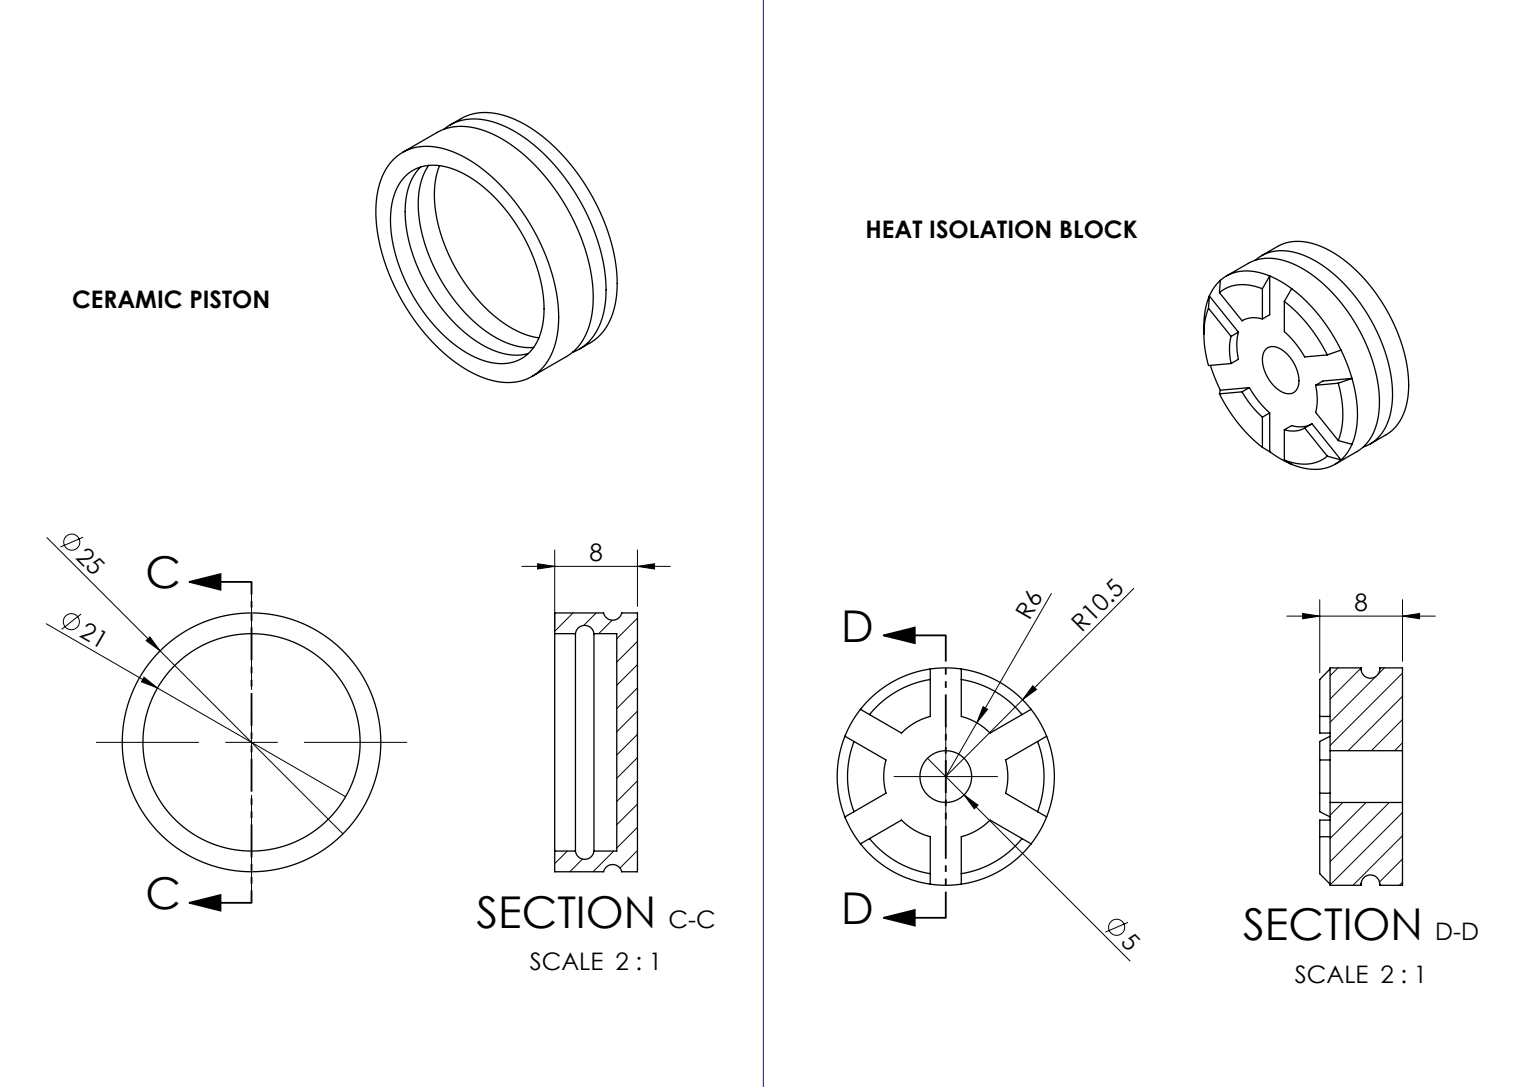
ISO-10303-21;
HEADER;
FILE_DESCRIPTION (('STEP AP214'),
    '1' );
FILE_NAME ('ceramic piston.step',
    '2026-09-24T10:28:59',
    ( '' ),
    ( '' ),
    'SwSTEP 2.0',
    'SolidWorks 2026',
    '' );
FILE_SCHEMA (( 'AUTOMOTIVE_DESIGN' ));
ENDSEC;

DATA;
#112=CARTESIAN_POINT ( 'NONE',  ( 0.000000000000000000, 0.000000000000000000, -4.000000000000000000 ) ) ;
#155=ORIENTED_EDGE ( 'NONE', *, *, #14955, .F. ) ;
#250=CARTESIAN_POINT ( 'NONE',  ( 0.000000000000000000, 0.000000000000000000, -9.600000000000001421 ) ) ;
#253=CARTESIAN_POINT ( 'NONE',  ( 0.000000000000000000, 0.000000000000000000, -9.600000000000001421 ) ) ;
#293=DIRECTION ( 'NONE',  ( 0.9237280213470681067, 0.3830490080632377170, 0.000000000000000000 ) ) ;
#316=CARTESIAN_POINT ( 'NONE',  ( 0.000000000000000000, 0.000000000000000000, -4.000000000000000000 ) ) ;
#333=DIRECTION ( 'NONE',  ( 1.000000000000000000, 0.000000000000000000, -0.000000000000000000 ) ) ;
#391=DIRECTION ( 'NONE',  ( 0.000000000000000000, 0.000000000000000000, 1.000000000000000000 ) ) ;
#452=ORIENTED_EDGE ( 'NONE', *, *, #3011, .F. ) ;
#524=DIRECTION ( 'NONE',  ( 1.000000000000000000, 0.000000000000000000, 0.000000000000000000 ) ) ;
#531=ORIENTED_EDGE ( 'NONE', *, *, #5477, .T. ) ;
#536=VECTOR ( 'NONE', #17608, 1000.000000000000000 ) ;
#599=STYLED_ITEM ( 'NONE', ( #6343 ), #8978 ) ;
#629=ADVANCED_FACE ( 'NONE', ( #5533 ), #13348, .F. ) ;
#659=EDGE_CURVE ( 'NONE', #16901, #17078, #11601, .T. ) ;
#709=ADVANCED_FACE ( 'NONE', ( #11224 ), #11887, .F. ) ;
#714=VERTEX_POINT ( 'NONE', #14072 ) ;
#715=ORIENTED_EDGE ( 'NONE', *, *, #7263, .T. ) ;
#770=CYLINDRICAL_SURFACE ( 'NONE', #14705, 12.50000000000000000 ) ;
#788=PRODUCT_DEFINITION_FORMATION_WITH_SPECIFIED_SOURCE ( 'ANY', '', #8245, .NOT_KNOWN. ) ;
#804=EDGE_CURVE ( 'NONE', #14976, #15476, #12782, .T. ) ;
#811=( NAMED_UNIT ( * ) SI_UNIT ( $, .STERADIAN. ) SOLID_ANGLE_UNIT ( ) );
#858=DIRECTION ( 'NONE',  ( -0.000000000000000000, -0.000000000000000000, -1.000000000000000000 ) ) ;
#922=DIRECTION ( 'NONE',  ( -1.000000000000000000, 0.000000000000000000, 0.000000000000000000 ) ) ;
#925=AXIS2_PLACEMENT_3D ( 'NONE', #16168, #3464, #2298 ) ;
#964=CIRCLE ( 'NONE', #17508, 10.50000000000000000 ) ;
#1034=VERTEX_POINT ( 'NONE', #3000 ) ;
#1048=PRODUCT_DEFINITION ( 'UNKNOWN', '', #788, #12463 ) ;
#1143=ORIENTED_EDGE ( 'NONE', *, *, #6595, .F. ) ;
#1148=VECTOR ( 'NONE', #6040, 1000.000000000000000 ) ;
#1152=CARTESIAN_POINT ( 'NONE',  ( 11.73134587110777005, 4.864722402403120149, -9.600000000000001421 ) ) ;
#1158=VERTEX_POINT ( 'NONE', #9063 ) ;
#1172=AXIS2_PLACEMENT_3D ( 'NONE', #8228, #13759, #1339 ) ;
#1199=CARTESIAN_POINT ( 'NONE',  ( 0.000000000000000000, 0.000000000000000000, -4.000000000000000000 ) ) ;
#1261=DIRECTION ( 'NONE',  ( 0.000000000000000000, 0.000000000000000000, 1.000000000000000000 ) ) ;
#1315=ORIENTED_EDGE ( 'NONE', *, *, #13930, .F. ) ;
#1339=DIRECTION ( 'NONE',  ( 1.000000000000000000, 0.000000000000000000, 0.000000000000000000 ) ) ;
#1365=CARTESIAN_POINT ( 'NONE',  ( 0.000000000000000000, 0.000000000000000000, -10.00000000000000000 ) ) ;
#1438=AXIS2_PLACEMENT_3D ( 'NONE', #2614, #17876, #10918 ) ;
#1444=CIRCLE ( 'NONE', #7818, 12.50000000000000000 ) ;
#1469=COLOUR_RGB ( '', 0.72549020, 0.75294118, 0.79215686) ;
#1475=EDGE_LOOP ( 'NONE', ( #10011, #4500, #155, #17294, #7332 ) ) ;
#1495=CYLINDRICAL_SURFACE ( 'NONE', #12703, 10.50000000000000000 ) ;
#1505=TOROIDAL_SURFACE ( 'NONE', #14826, 10.40000000000000036, 0.9000000000000003553 ) ;
#1527=DIRECTION ( 'NONE',  ( 1.000000000000000000, 0.000000000000000000, 0.000000000000000000 ) ) ;
#1538=ADVANCED_FACE ( 'NONE', ( #6383 ), #1505, .F. ) ;
#1541=CIRCLE ( 'NONE', #11662, 10.50000000000000000 ) ;
#1555=ORIENTED_EDGE ( 'NONE', *, *, #12558, .F. ) ;
#1556=AXIS2_PLACEMENT_3D ( 'NONE', #12533, #15688, #5624 ) ;
#1570=VERTEX_POINT ( 'NONE', #6290 ) ;
#1706=FACE_OUTER_BOUND ( 'NONE', #10911, .T. ) ;
#1743=ADVANCED_FACE ( 'NONE', ( #15891 ), #14883, .T. ) ;
#1830=LINE ( 'NONE', #17063, #3240 ) ;
#1846=EDGE_CURVE ( 'NONE', #16993, #17950, #4103, .T. ) ;
#1863=AXIS2_PLACEMENT_3D ( 'NONE', #15659, #6311, #2165 ) ;
#1877=CARTESIAN_POINT ( 'NONE',  ( 12.50000000000000000, 1.530808498934191521E-15, -10.47749643873921244 ) ) ;
#1897=CARTESIAN_POINT ( 'NONE',  ( 0.000000000000000000, 0.000000000000000000, -12.00000000000000000 ) ) ;
#1937=EDGE_CURVE ( 'NONE', #16345, #6066, #10175, .T. ) ;
#1962=DIRECTION ( 'NONE',  ( -5.026720092345836698E-22, 4.581671729415424240E-22, -1.000000000000000000 ) ) ;
#1978=ORIENTED_EDGE ( 'NONE', *, *, #804, .F. ) ;
#2009=AXIS2_PLACEMENT_3D ( 'NONE', #10405, #10657, #10838 ) ;
#2016=EDGE_LOOP ( 'NONE', ( #5308, #3767, #12168, #12352, #15309 ) ) ;
#2054=CIRCLE ( 'NONE', #4054, 10.50000000000000000 ) ;
#2086=ORIENTED_EDGE ( 'NONE', *, *, #12227, .F. ) ;
#2089=VERTEX_POINT ( 'NONE', #7177 ) ;
#2101=EDGE_CURVE ( 'NONE', #9766, #6169, #5832, .T. ) ;
#2103=( NAMED_UNIT ( * ) PLANE_ANGLE_UNIT ( ) SI_UNIT ( $, .RADIAN. ) );
#2146=EDGE_CURVE ( 'NONE', #9766, #2089, #1830, .T. ) ;
#2165=DIRECTION ( 'NONE',  ( -1.000000000000000000, 0.000000000000000000, 0.000000000000000000 ) ) ;
#2195=( NAMED_UNIT ( * ) PLANE_ANGLE_UNIT ( ) SI_UNIT ( $, .RADIAN. ) );
#2230=DIRECTION ( 'NONE',  ( 5.026720092345836698E-22, -4.581671729415424240E-22, 1.000000000000000000 ) ) ;
#2298=DIRECTION ( 'NONE',  ( -1.000000000000000000, 0.000000000000000000, 0.000000000000000000 ) ) ;
#2338=CARTESIAN_POINT ( 'NONE',  ( 0.000000000000000000, 0.000000000000000000, -4.000000000000000000 ) ) ;
#2471=EDGE_CURVE ( 'NONE', #1158, #1034, #7607, .T. ) ;
#2482=CARTESIAN_POINT ( 'NONE',  ( 0.000000000000000000, 0.000000000000000000, -10.00000000000000000 ) ) ;
#2494=SURFACE_STYLE_FILL_AREA ( #4027 ) ;
#2598=DIRECTION ( 'NONE',  ( 0.9237280213470682178, 0.3830490080632377170, 0.000000000000000000 ) ) ;
#2613=DIRECTION ( 'NONE',  ( -0.3830490080632376615, 0.9237280213470682178, 0.000000000000000000 ) ) ;
#2614=CARTESIAN_POINT ( 'NONE',  ( 0.000000000000000000, 0.000000000000000000, -9.600000000000001421 ) ) ;
#2623=ADVANCED_FACE ( 'NONE', ( #12156 ), #5002, .T. ) ;
#2627=STYLED_ITEM ( 'NONE', ( #17931 ), #11433 ) ;
#2632=AXIS2_PLACEMENT_3D ( 'NONE', #112, #391, #5897 ) ;
#2684=AXIS2_PLACEMENT_3D ( 'NONE', #253, #10021, #16757 ) ;
#2690=EDGE_CURVE ( 'NONE', #6877, #15184, #9894, .T. ) ;
#2691=CARTESIAN_POINT ( 'NONE',  ( 10.50000000000000000, 1.285879139104720831E-15, -4.000000000000000000 ) ) ;
#2706=DIRECTION ( 'NONE',  ( -1.000000000000000000, 0.000000000000000000, 0.000000000000000000 ) ) ;
#2741=LINE ( 'NONE', #8262, #13559 ) ;
#2764=SURFACE_STYLE_USAGE ( .BOTH. , #8017 ) ;
#2788=ADVANCED_FACE ( 'NONE', ( #9518 ), #16296, .F. ) ;
#2793=CARTESIAN_POINT ( 'NONE',  ( -11.54660026683835383, -4.788112600790469742, -10.47749643873921244 ) ) ;
#2837=ORIENTED_EDGE ( 'NONE', *, *, #804, .T. ) ;
#2900=( GEOMETRIC_REPRESENTATION_CONTEXT ( 3 ) GLOBAL_UNCERTAINTY_ASSIGNED_CONTEXT ( ( #12605 ) ) GLOBAL_UNIT_ASSIGNED_CONTEXT ( ( #13555, #12455, #3862 ) ) REPRESENTATION_CONTEXT ( 'NONE', 'WORKASPACE' ) );
#2946=DIRECTION ( 'NONE',  ( 1.000000000000000000, -4.440892098500626162E-15, 0.000000000000000000 ) ) ;
#3000=CARTESIAN_POINT ( 'NONE',  ( 11.54660026683835206, 4.788112600790471518, -10.47749643873921244 ) ) ;
#3011=EDGE_CURVE ( 'NONE', #15476, #16993, #13400, .T. ) ;
#3190=EDGE_LOOP ( 'NONE', ( #4795, #17103, #11231, #9291, #13094, #3504 ) ) ;
#3233=ORIENTED_EDGE ( 'NONE', *, *, #17773, .F. ) ;
#3240=VECTOR ( 'NONE', #6438, 1000.000000000000000 ) ;
#3256=ORIENTED_EDGE ( 'NONE', *, *, #16158, .T. ) ;
#3285=FACE_OUTER_BOUND ( 'NONE', #8751, .T. ) ;
#3349=CARTESIAN_POINT ( 'NONE',  ( 11.54660026683835206, 4.788112600790471518, -8.722503561260788629 ) ) ;
#3358=CARTESIAN_POINT ( 'NONE',  ( 8.472608240843633681E-22, -7.722472891792491889E-22, -7.794427190999915211 ) ) ;
#3382=CARTESIAN_POINT ( 'NONE',  ( -10.89999065189540772, -4.519978295146205305, -9.600000000000001421 ) ) ;
#3393=CIRCLE ( 'NONE', #8898, 12.50000000000000000 ) ;
#3430=AXIS2_PLACEMENT_3D ( 'NONE', #1199, #10952, #8080 ) ;
#3464=DIRECTION ( 'NONE',  ( -0.000000000000000000, -0.000000000000000000, -1.000000000000000000 ) ) ;
#3504=ORIENTED_EDGE ( 'NONE', *, *, #6011, .T. ) ;
#3531=AXIS2_PLACEMENT_3D ( 'NONE', #2482, #10701, #17662 ) ;
#3556=EDGE_CURVE ( 'NONE', #17384, #13349, #3393, .T. ) ;
#3575=AXIS2_PLACEMENT_3D ( 'NONE', #5095, #17575, #9272 ) ;
#3606=ORIENTED_EDGE ( 'NONE', *, *, #9596, .T. ) ;
#3640=VERTEX_POINT ( 'NONE', #3382 ) ;
#3750=AXIS2_PLACEMENT_3D ( 'NONE', #10192, #1962, #10363 ) ;
#3767=ORIENTED_EDGE ( 'NONE', *, *, #5434, .T. ) ;
#3784=( GEOMETRIC_REPRESENTATION_CONTEXT ( 3 ) GLOBAL_UNCERTAINTY_ASSIGNED_CONTEXT ( ( #4445 ) ) GLOBAL_UNIT_ASSIGNED_CONTEXT ( ( #13509, #2103, #811 ) ) REPRESENTATION_CONTEXT ( 'NONE', 'WORKASPACE' ) );
#3793=ORIENTED_EDGE ( 'NONE', *, *, #2471, .T. ) ;
#3840=CIRCLE ( 'NONE', #8463, 0.9000000000000011324 ) ;
#3849=DIRECTION ( 'NONE',  ( -0.9979201627913402151, 0.06446199418653550395, 5.311609029246448998E-22 ) ) ;
#3860=ORIENTED_EDGE ( 'NONE', *, *, #2101, .T. ) ;
#3862=( NAMED_UNIT ( * ) SI_UNIT ( $, .STERADIAN. ) SOLID_ANGLE_UNIT ( ) );
#3888=DIRECTION ( 'NONE',  ( -0.000000000000000000, -0.000000000000000000, -1.000000000000000000 ) ) ;
#3911=CARTESIAN_POINT ( 'NONE',  ( 0.000000000000000000, 0.000000000000000000, -8.722503561260788629 ) ) ;
#3924=EDGE_CURVE ( 'NONE', #6169, #8696, #9457, .T. ) ;
#3984=ADVANCED_FACE ( 'NONE', ( #16284 ), #770, .T. ) ;
#4010=CIRCLE ( 'NONE', #10365, 0.9000000000000011324 ) ;
#4024=CARTESIAN_POINT ( 'NONE',  ( 0.000000000000000000, 0.000000000000000000, -8.722503561260788629 ) ) ;
#4027=FILL_AREA_STYLE ('',( #16293 ) ) ;
#4054=AXIS2_PLACEMENT_3D ( 'NONE', #8842, #15368, #5926 ) ;
#4057=CARTESIAN_POINT ( 'NONE',  ( 0.000000000000000000, 0.000000000000000000, -4.000000000000000000 ) ) ;
#4097=CIRCLE ( 'NONE', #17745, 0.9000000000000003553 ) ;
#4103=CIRCLE ( 'NONE', #9881, 10.50000000000000000 ) ;
#4195=CARTESIAN_POINT ( 'NONE',  ( 0.000000000000000000, 0.000000000000000000, -9.600000000000001421 ) ) ;
#4276=ORIENTED_EDGE ( 'NONE', *, *, #5477, .F. ) ;
#4308=DIRECTION ( 'NONE',  ( 1.000000000000000000, 0.000000000000000000, 0.000000000000000000 ) ) ;
#4339=ORIENTED_EDGE ( 'NONE', *, *, #5350, .T. ) ;
#4393=EDGE_LOOP ( 'NONE', ( #8466, #15017, #11576, #7109, #5872 ) ) ;
#4424=DIRECTION ( 'NONE',  ( 0.000000000000000000, 0.000000000000000000, 1.000000000000000000 ) ) ;
#4432=CIRCLE ( 'NONE', #11963, 10.50000000000000000 ) ;
#4445=UNCERTAINTY_MEASURE_WITH_UNIT (LENGTH_MEASURE( 1.000000000000000082E-05 ), #13509, 'distance_accuracy_value', 'NONE');
#4491=FACE_OUTER_BOUND ( 'NONE', #10765, .T. ) ;
#4495=CARTESIAN_POINT ( 'NONE',  ( -10.47816170930907553, 0.6768509389586230274, -7.794427190999915211 ) ) ;
#4500=ORIENTED_EDGE ( 'NONE', *, *, #8547, .T. ) ;
#4630=PLANE ( 'NONE',  #16310 ) ;
#4653=DIRECTION ( 'NONE',  ( -1.000000000000000000, -1.065814103640150279E-14, 0.000000000000000000 ) ) ;
#4720=EDGE_CURVE ( 'NONE', #714, #6066, #17381, .T. ) ;
#4795=ORIENTED_EDGE ( 'NONE', *, *, #12262, .F. ) ;
#4811=APPLICATION_CONTEXT ( 'automotive_design' ) ;
#4924=CARTESIAN_POINT ( 'NONE',  ( 1.746467850512308208E-21, -1.591841644184202181E-21, -6.005572809000082835 ) ) ;
#5002=CYLINDRICAL_SURFACE ( 'NONE', #7017, 12.50000000000000000 ) ;
#5095=CARTESIAN_POINT ( 'NONE',  ( 0.000000000000000000, 0.000000000000000000, 0.000000000000000000 ) ) ;
#5116=CARTESIAN_POINT ( 'NONE',  ( 12.50000000000000000, 1.530808498934191521E-15, -4.000000000000000000 ) ) ;
#5148=SURFACE_STYLE_FILL_AREA ( #6606 ) ;
#5160=DIRECTION ( 'NONE',  ( 0.06446199418653537905, 0.9979201627913403261, 4.248110196704583871E-22 ) ) ;
#5184=PLANE ( 'NONE',  #3531 ) ;
#5252=AXIS2_PLACEMENT_3D ( 'NONE', #1365, #6890, #12419 ) ;
#5261=DIRECTION ( 'NONE',  ( -0.9979201627913402151, 0.06446199418653550395, 5.311609029246448998E-22 ) ) ;
#5267=AXIS2_PLACEMENT_3D ( 'NONE', #9775, #6898, #16518 ) ;
#5308=ORIENTED_EDGE ( 'NONE', *, *, #8547, .F. ) ;
#5350=EDGE_CURVE ( 'NONE', #1158, #3640, #14742, .T. ) ;
#5434=EDGE_CURVE ( 'NONE', #3640, #6169, #4010, .T. ) ;
#5457=AXIS2_PLACEMENT_3D ( 'NONE', #9421, #8920, #4653 ) ;
#5477=EDGE_CURVE ( 'NONE', #17078, #16901, #8353, .T. ) ;
#5533=FACE_OUTER_BOUND ( 'NONE', #2016, .T. ) ;
#5539=CIRCLE ( 'NONE', #17468, 0.9000000000000011324 ) ;
#5554=AXIS2_PLACEMENT_3D ( 'NONE', #8563, #16731, #2946 ) ;
#5624=DIRECTION ( 'NONE',  ( -1.000000000000000000, 0.000000000000000000, 0.000000000000000000 ) ) ;
#5636=ORIENTED_EDGE ( 'NONE', *, *, #6443, .F. ) ;
#5643=LINE ( 'NONE', #8651, #15902 ) ;
#5706=ORIENTED_EDGE ( 'NONE', *, *, #8457, .T. ) ;
#5756=ORIENTED_EDGE ( 'NONE', *, *, #16630, .T. ) ;
#5763=CARTESIAN_POINT ( 'NONE',  ( -10.47816170930907553, 0.6768509389586230274, -6.005572809000082835 ) ) ;
#5802=CIRCLE ( 'NONE', #12188, 12.50000000000000000 ) ;
#5832=CIRCLE ( 'NONE', #8171, 12.50000000000000000 ) ;
#5835=PRODUCT_CONTEXT ( 'NONE', #13620, 'mechanical' ) ;
#5872=ORIENTED_EDGE ( 'NONE', *, *, #9666, .F. ) ;
#5897=DIRECTION ( 'NONE',  ( 1.000000000000000000, 0.000000000000000000, 0.000000000000000000 ) ) ;
#5918=DIRECTION ( 'NONE',  ( 0.9979201627913403261, -0.06446199418653547619, 0.000000000000000000 ) ) ;
#5926=DIRECTION ( 'NONE',  ( 1.000000000000000000, 0.000000000000000000, 0.000000000000000000 ) ) ;
#5953=ADVANCED_FACE ( 'NONE', ( #6627 ), #16356, .F. ) ;
#6011=EDGE_CURVE ( 'NONE', #13121, #11972, #7798, .T. ) ;
#6025=ORIENTED_EDGE ( 'NONE', *, *, #9596, .F. ) ;
#6030=FACE_OUTER_BOUND ( 'NONE', #15171, .T. ) ;
#6040=DIRECTION ( 'NONE',  ( -0.000000000000000000, -0.000000000000000000, -1.000000000000000000 ) ) ;
#6066=VERTEX_POINT ( 'NONE', #7458 ) ;
#6140=CARTESIAN_POINT ( 'NONE',  ( -12.50000000000000000, 0.000000000000000000, -4.000000000000000000 ) ) ;
#6165=CARTESIAN_POINT ( 'NONE',  ( -12.50000000000000000, 0.000000000000000000, -10.47749643873921244 ) ) ;
#6169=VERTEX_POINT ( 'NONE', #2793 ) ;
#6235=EDGE_CURVE ( 'NONE', #1570, #2089, #17079, .T. ) ;
#6254=( LENGTH_UNIT ( ) NAMED_UNIT ( * ) SI_UNIT ( .MILLI., .METRE. ) );
#6290=CARTESIAN_POINT ( 'NONE',  ( -12.50000000000000000, 0.000000000000000000, -12.00000000000000000 ) ) ;
#6311=DIRECTION ( 'NONE',  ( -0.000000000000000000, -0.000000000000000000, -1.000000000000000000 ) ) ;
#6343=PRESENTATION_STYLE_ASSIGNMENT (( #6528 ) ) ;
#6383=FACE_OUTER_BOUND ( 'NONE', #3190, .T. ) ;
#6438=DIRECTION ( 'NONE',  ( -0.000000000000000000, -0.000000000000000000, -1.000000000000000000 ) ) ;
#6443=EDGE_CURVE ( 'NONE', #8696, #1570, #5643, .T. ) ;
#6457=CARTESIAN_POINT ( 'NONE',  ( 10.37836969302994028, -0.6704047395399680420, -6.899999999999998579 ) ) ;
#6465=DIRECTION ( 'NONE',  ( 1.000000000000000000, 0.000000000000000000, 0.000000000000000000 ) ) ;
#6509=ADVANCED_FACE ( 'NONE', ( #16821 ), #1495, .F. ) ;
#6528=SURFACE_STYLE_USAGE ( .BOTH. , #12043 ) ;
#6540=DIRECTION ( 'NONE',  ( 0.000000000000000000, 0.000000000000000000, 1.000000000000000000 ) ) ;
#6541=DIRECTION ( 'NONE',  ( 0.3830490080632377725, -0.9237280213470682178, 0.000000000000000000 ) ) ;
#6595=EDGE_CURVE ( 'NONE', #15658, #16993, #9799, .T. ) ;
#6606=FILL_AREA_STYLE ('',( #16068 ) ) ;
#6627=FACE_OUTER_BOUND ( 'NONE', #4393, .T. ) ;
#6712=CARTESIAN_POINT ( 'NONE',  ( 1.746467850512308208E-21, -1.591841644184202181E-21, -6.005572809000082835 ) ) ;
#6719=CARTESIAN_POINT ( 'NONE',  ( 10.50000000000000000, 1.285879139104720831E-15, -7.794427190999915211 ) ) ;
#6731=CIRCLE ( 'NONE', #14277, 0.9000000000000003553 ) ;
#6794=VERTEX_POINT ( 'NONE', #8518 ) ;
#6877=VERTEX_POINT ( 'NONE', #3349 ) ;
#6890=DIRECTION ( 'NONE',  ( 0.000000000000000000, 0.000000000000000000, 1.000000000000000000 ) ) ;
#6898=DIRECTION ( 'NONE',  ( 0.000000000000000000, 0.000000000000000000, 1.000000000000000000 ) ) ;
#7017=AXIS2_PLACEMENT_3D ( 'NONE', #17650, #11798, #14721 ) ;
#7109=ORIENTED_EDGE ( 'NONE', *, *, #4720, .F. ) ;
#7135=DIRECTION ( 'NONE',  ( 0.000000000000000000, 0.000000000000000000, 1.000000000000000000 ) ) ;
#7177=CARTESIAN_POINT ( 'NONE',  ( 12.50000000000000000, 1.530808498934191521E-15, -12.00000000000000000 ) ) ;
#7204=DIRECTION ( 'NONE',  ( 0.000000000000000000, 0.000000000000000000, 1.000000000000000000 ) ) ;
#7219=ADVANCED_FACE ( 'NONE', ( #16405 ), #15036, .F. ) ;
#7224=PLANE ( 'NONE',  #13964 ) ;
#7242=ADVANCED_FACE ( 'NONE', ( #9568 ), #15026, .T. ) ;
#7263=EDGE_CURVE ( 'NONE', #2089, #1570, #16493, .T. ) ;
#7273=COLOUR_RGB ( '', 0.72549020, 0.75294118, 0.79215686) ;
#7279=CARTESIAN_POINT ( 'NONE',  ( 0.000000000000000000, 0.000000000000000000, -4.000000000000000000 ) ) ;
#7332=ORIENTED_EDGE ( 'NONE', *, *, #3556, .F. ) ;
#7375=DIRECTION ( 'NONE',  ( 0.000000000000000000, 0.000000000000000000, 1.000000000000000000 ) ) ;
#7454=CARTESIAN_POINT ( 'NONE',  ( 10.47816170930907553, -0.6768509389586216951, -7.794427190999915211 ) ) ;
#7458=CARTESIAN_POINT ( 'NONE',  ( -10.50000000000000000, 0.000000000000000000, -10.00000000000000000 ) ) ;
#7476=ORIENTED_EDGE ( 'NONE', *, *, #1846, .T. ) ;
#7507=LINE ( 'NONE', #6140, #1148 ) ;
#7517=EDGE_CURVE ( 'NONE', #16901, #13349, #17597, .T. ) ;
#7541=VECTOR ( 'NONE', #13295, 1000.000000000000000 ) ;
#7569=CARTESIAN_POINT ( 'NONE',  ( -10.37836969302994028, 0.6704047395399693743, -6.899999999999998579 ) ) ;
#7585=AXIS2_PLACEMENT_3D ( 'NONE', #11276, #8311, #11182 ) ;
#7607=CIRCLE ( 'NONE', #7891, 0.9000000000000011324 ) ;
#7740=ORIENTED_EDGE ( 'NONE', *, *, #2146, .T. ) ;
#7744=DIRECTION ( 'NONE',  ( -1.000000000000000000, 0.000000000000000000, 0.000000000000000000 ) ) ;
#7780=ORIENTED_EDGE ( 'NONE', *, *, #7517, .F. ) ;
#7798=CIRCLE ( 'NONE', #15320, 10.50000000000000000 ) ;
#7818=AXIS2_PLACEMENT_3D ( 'NONE', #11359, #16928, #4308 ) ;
#7880=EDGE_LOOP ( 'NONE', ( #17660, #1978 ) ) ;
#7891=AXIS2_PLACEMENT_3D ( 'NONE', #9169, #6541, #13343 ) ;
#7946=EDGE_LOOP ( 'NONE', ( #11758, #4339, #1555, #2086, #11320 ) ) ;
#7961=ORIENTED_EDGE ( 'NONE', *, *, #7517, .T. ) ;
#7968=CARTESIAN_POINT ( 'NONE',  ( -11.73134587110777005, -4.864722402403119261, -9.600000000000001421 ) ) ;
#7979=EDGE_LOOP ( 'NONE', ( #7780, #4276, #17656, #14589, #16002 ) ) ;
#7993=CARTESIAN_POINT ( 'NONE',  ( 8.472608240843633681E-22, -7.722472891792491889E-22, -7.794427190999915211 ) ) ;
#8010=DIRECTION ( 'NONE',  ( -1.000000000000000000, 0.000000000000000000, 0.000000000000000000 ) ) ;
#8017=SURFACE_SIDE_STYLE ('',( #2494 ) ) ;
#8080=DIRECTION ( 'NONE',  ( -1.000000000000000000, 0.000000000000000000, 0.000000000000000000 ) ) ;
#8125=DIRECTION ( 'NONE',  ( 0.3830490080632377725, -0.9237280213470682178, 0.000000000000000000 ) ) ;
#8141=CARTESIAN_POINT ( 'NONE',  ( 0.000000000000000000, 0.000000000000000000, -4.000000000000000000 ) ) ;
#8171=AXIS2_PLACEMENT_3D ( 'NONE', #11493, #8803, #11305 ) ;
#8228=CARTESIAN_POINT ( 'NONE',  ( 0.000000000000000000, 0.000000000000000000, -12.00000000000000000 ) ) ;
#8245=PRODUCT ( 'ceramic piston', 'ceramic piston', '', ( #5835 ) ) ;
#8262=CARTESIAN_POINT ( 'NONE',  ( 10.50000000000000000, 1.285879139104720831E-15, -4.000000000000000000 ) ) ;
#8311=DIRECTION ( 'NONE',  ( 0.000000000000000000, 0.000000000000000000, 1.000000000000000000 ) ) ;
#8353=CIRCLE ( 'NONE', #8931, 12.50000000000000000 ) ;
#8457=EDGE_CURVE ( 'NONE', #15476, #14976, #1541, .T. ) ;
#8463=AXIS2_PLACEMENT_3D ( 'NONE', #1152, #8125, #2598 ) ;
#8466=ORIENTED_EDGE ( 'NONE', *, *, #6011, .F. ) ;
#8470=DIRECTION ( 'NONE',  ( -1.000000000000000000, 0.000000000000000000, 0.000000000000000000 ) ) ;
#8485=CARTESIAN_POINT ( 'NONE',  ( 0.000000000000000000, 0.000000000000000000, -12.00000000000000000 ) ) ;
#8518=CARTESIAN_POINT ( 'NONE',  ( 10.50000000000000000, 1.285879139104720831E-15, -6.005572809000082835 ) ) ;
#8539=DIRECTION ( 'NONE',  ( 0.9237280213470681067, 0.3830490080632377170, 0.000000000000000000 ) ) ;
#8547=EDGE_CURVE ( 'NONE', #3640, #1158, #13691, .T. ) ;
#8563=CARTESIAN_POINT ( 'NONE',  ( 0.000000000000000000, 0.000000000000000000, -10.47749643873921244 ) ) ;
#8625=CYLINDRICAL_SURFACE ( 'NONE', #11968, 10.50000000000000000 ) ;
#8651=CARTESIAN_POINT ( 'NONE',  ( -12.50000000000000000, 0.000000000000000000, -4.000000000000000000 ) ) ;
#8696=VERTEX_POINT ( 'NONE', #6165 ) ;
#8709=MECHANICAL_DESIGN_GEOMETRIC_PRESENTATION_REPRESENTATION('',(#2627),#2900);
#8725=FACE_OUTER_BOUND ( 'NONE', #10604, .T. ) ;
#8746=EDGE_CURVE ( 'NONE', #16745, #13121, #4432, .T. ) ;
#8751=EDGE_LOOP ( 'NONE', ( #17194, #2837, #12747, #1143, #12287 ) ) ;
#8803=DIRECTION ( 'NONE',  ( -0.000000000000000000, -0.000000000000000000, -1.000000000000000000 ) ) ;
#8816=DIRECTION ( 'NONE',  ( -0.000000000000000000, -0.000000000000000000, -1.000000000000000000 ) ) ;
#8842=CARTESIAN_POINT ( 'NONE',  ( 8.472608240843633681E-22, -7.722472891792491889E-22, -7.794427190999915211 ) ) ;
#8877=ORIENTED_EDGE ( 'NONE', *, *, #5350, .F. ) ;
#8898=AXIS2_PLACEMENT_3D ( 'NONE', #4024, #7204, #12449 ) ;
#8920=DIRECTION ( 'NONE',  ( 5.026720092345836698E-22, -4.581671729415424240E-22, 1.000000000000000000 ) ) ;
#8931=AXIS2_PLACEMENT_3D ( 'NONE', #8141, #1261, #1527 ) ;
#8978=ADVANCED_BREP_SHAPE_REPRESENTATION ( '', ( #11433, #3575 ), #3784 ) ;
#9063=CARTESIAN_POINT ( 'NONE',  ( 10.89999065189540772, 4.519978295146206193, -9.600000000000001421 ) ) ;
#9071=SHAPE_REPRESENTATION_RELATIONSHIP ( 'NONE' , 'NONE' ,  #16332, #8978 ) ;
#9126=DIRECTION ( 'NONE',  ( 0.000000000000000000, 0.000000000000000000, 1.000000000000000000 ) ) ;
#9169=CARTESIAN_POINT ( 'NONE',  ( 11.73134587110777005, 4.864722402403120149, -9.600000000000001421 ) ) ;
#9172=UNCERTAINTY_MEASURE_WITH_UNIT (LENGTH_MEASURE( 1.000000000000000082E-05 ), #6254, 'distance_accuracy_value', 'NONE');
#9180=EDGE_CURVE ( 'NONE', #17078, #15184, #7507, .T. ) ;
#9272=DIRECTION ( 'NONE',  ( 1.000000000000000000, 0.000000000000000000, 0.000000000000000000 ) ) ;
#9275=( GEOMETRIC_REPRESENTATION_CONTEXT ( 3 ) GLOBAL_UNCERTAINTY_ASSIGNED_CONTEXT ( ( #9172 ) ) GLOBAL_UNIT_ASSIGNED_CONTEXT ( ( #6254, #2195, #15970 ) ) REPRESENTATION_CONTEXT ( 'NONE', 'WORKASPACE' ) );
#9291=ORIENTED_EDGE ( 'NONE', *, *, #17773, .T. ) ;
#9421=CARTESIAN_POINT ( 'NONE',  ( 1.746467850512308208E-21, -1.591841644184202181E-21, -6.005572809000082835 ) ) ;
#9423=CARTESIAN_POINT ( 'NONE',  ( 0.000000000000000000, 0.000000000000000000, -4.000000000000000000 ) ) ;
#9457=CIRCLE ( 'NONE', #10888, 12.50000000000000000 ) ;
#9518=FACE_OUTER_BOUND ( 'NONE', #11290, .T. ) ;
#9568=FACE_OUTER_BOUND ( 'NONE', #10087, .T. ) ;
#9596=EDGE_CURVE ( 'NONE', #8696, #1034, #1444, .T. ) ;
#9666=EDGE_CURVE ( 'NONE', #11972, #714, #2054, .T. ) ;
#9672=EDGE_LOOP ( 'NONE', ( #13955, #12949, #1315, #10879, #13886 ) ) ;
#9680=DIRECTION ( 'NONE',  ( 0.000000000000000000, 0.000000000000000000, 1.000000000000000000 ) ) ;
#9766=VERTEX_POINT ( 'NONE', #1877 ) ;
#9775=CARTESIAN_POINT ( 'NONE',  ( 0.000000000000000000, 0.000000000000000000, -8.722503561260788629 ) ) ;
#9799=CIRCLE ( 'NONE', #5457, 10.50000000000000000 ) ;
#9879=CARTESIAN_POINT ( 'NONE',  ( -12.50000000000000000, 0.000000000000000000, -4.000000000000000000 ) ) ;
#9881=AXIS2_PLACEMENT_3D ( 'NONE', #6712, #13612, #16512 ) ;
#9894=CIRCLE ( 'NONE', #5267, 12.50000000000000000 ) ;
#9902=DIRECTION ( 'NONE',  ( -0.000000000000000000, -0.000000000000000000, -1.000000000000000000 ) ) ;
#9944=ORIENTED_EDGE ( 'NONE', *, *, #12597, .T. ) ;
#10011=ORIENTED_EDGE ( 'NONE', *, *, #12558, .T. ) ;
#10021=DIRECTION ( 'NONE',  ( 0.000000000000000000, 0.000000000000000000, 1.000000000000000000 ) ) ;
#10087=EDGE_LOOP ( 'NONE', ( #16850, #3860, #17086, #11688, #14910 ) ) ;
#10175=CIRCLE ( 'NONE', #5252, 10.50000000000000000 ) ;
#10192=CARTESIAN_POINT ( 'NONE',  ( 8.472608240843633681E-22, -7.722472891792491889E-22, -7.794427190999915211 ) ) ;
#10336=ORIENTED_EDGE ( 'NONE', *, *, #1937, .T. ) ;
#10355=DIRECTION ( 'NONE',  ( -0.06446199418653550395, -0.9979201627913403261, -4.248110196704583871E-22 ) ) ;
#10363=DIRECTION ( 'NONE',  ( 1.000000000000000000, 0.000000000000000000, 0.000000000000000000 ) ) ;
#10365=AXIS2_PLACEMENT_3D ( 'NONE', #7968, #2613, #17706 ) ;
#10380=CYLINDRICAL_SURFACE ( 'NONE', #1863, 10.50000000000000000 ) ;
#10405=CARTESIAN_POINT ( 'NONE',  ( 0.000000000000000000, 0.000000000000000000, -9.600000000000001421 ) ) ;
#10498=CARTESIAN_POINT ( 'NONE',  ( 10.50000000000000000, 1.285879139104720831E-15, -4.000000000000000000 ) ) ;
#10589=CARTESIAN_POINT ( 'NONE',  ( 1.746467850512308208E-21, -1.591841644184202181E-21, -6.005572809000082835 ) ) ;
#10604=EDGE_LOOP ( 'NONE', ( #531, #11943 ) ) ;
#10623=CARTESIAN_POINT ( 'NONE',  ( 0.000000000000000000, 0.000000000000000000, -10.47749643873921244 ) ) ;
#10657=DIRECTION ( 'NONE',  ( 0.000000000000000000, 0.000000000000000000, 1.000000000000000000 ) ) ;
#10659=CARTESIAN_POINT ( 'NONE',  ( -11.73134587110777005, -4.864722402403119261, -9.600000000000001421 ) ) ;
#10701=DIRECTION ( 'NONE',  ( 0.000000000000000000, 0.000000000000000000, 1.000000000000000000 ) ) ;
#10765=EDGE_LOOP ( 'NONE', ( #15447, #17309 ) ) ;
#10838=DIRECTION ( 'NONE',  ( 1.000000000000000000, 0.000000000000000000, 0.000000000000000000 ) ) ;
#10879=ORIENTED_EDGE ( 'NONE', *, *, #4720, .T. ) ;
#10888=AXIS2_PLACEMENT_3D ( 'NONE', #10623, #16196, #11819 ) ;
#10911=EDGE_LOOP ( 'NONE', ( #8877, #3793, #6025, #14457, #11378 ) ) ;
#10918=DIRECTION ( 'NONE',  ( 0.9237280213470681067, 0.3830490080632377170, 0.000000000000000000 ) ) ;
#10952=DIRECTION ( 'NONE',  ( -0.000000000000000000, -0.000000000000000000, -1.000000000000000000 ) ) ;
#11031=AXIS2_PLACEMENT_3D ( 'NONE', #250, #16486, #13761 ) ;
#11057=CARTESIAN_POINT ( 'NONE',  ( 12.50000000000000000, 1.530808498934191521E-15, -4.000000000000000000 ) ) ;
#11182=DIRECTION ( 'NONE',  ( 1.000000000000000000, 0.000000000000000000, 0.000000000000000000 ) ) ;
#11224=FACE_OUTER_BOUND ( 'NONE', #7946, .T. ) ;
#11231=ORIENTED_EDGE ( 'NONE', *, *, #16302, .T. ) ;
#11276=CARTESIAN_POINT ( 'NONE',  ( 0.000000000000000000, 0.000000000000000000, -10.00000000000000000 ) ) ;
#11290=EDGE_LOOP ( 'NONE', ( #7476, #17509, #13360, #14481, #3233, #15733 ) ) ;
#11305=DIRECTION ( 'NONE',  ( 1.000000000000000000, 0.000000000000000000, 0.000000000000000000 ) ) ;
#11320=ORIENTED_EDGE ( 'NONE', *, *, #2690, .F. ) ;
#11359=CARTESIAN_POINT ( 'NONE',  ( 0.000000000000000000, 0.000000000000000000, -10.47749643873921244 ) ) ;
#11378=ORIENTED_EDGE ( 'NONE', *, *, #5434, .F. ) ;
#11433=MANIFOLD_SOLID_BREP ( 'Cavity1', #15959 ) ;
#11442=ORIENTED_EDGE ( 'NONE', *, *, #13539, .F. ) ;
#11493=CARTESIAN_POINT ( 'NONE',  ( 0.000000000000000000, 0.000000000000000000, -10.47749643873921244 ) ) ;
#11506=CARTESIAN_POINT ( 'NONE',  ( -10.50000000000000000, -1.591841644184202181E-21, -6.005572809000082835 ) ) ;
#11576=ORIENTED_EDGE ( 'NONE', *, *, #12652, .F. ) ;
#11601=CIRCLE ( 'NONE', #2632, 12.50000000000000000 ) ;
#11630=CARTESIAN_POINT ( 'NONE',  ( -10.50000000000000000, 0.000000000000000000, -4.000000000000000000 ) ) ;
#11632=CIRCLE ( 'NONE', #7585, 10.50000000000000000 ) ;
#11638=CARTESIAN_POINT ( 'NONE',  ( 10.50000000000000000, 1.285879139104720831E-15, -10.00000000000000000 ) ) ;
#11662=AXIS2_PLACEMENT_3D ( 'NONE', #2338, #9126, #14665 ) ;
#11688=ORIENTED_EDGE ( 'NONE', *, *, #6443, .T. ) ;
#11758=ORIENTED_EDGE ( 'NONE', *, *, #14955, .T. ) ;
#11798=DIRECTION ( 'NONE',  ( -0.000000000000000000, -0.000000000000000000, -1.000000000000000000 ) ) ;
#11819=DIRECTION ( 'NONE',  ( 1.000000000000000000, 3.552713678800500929E-15, 0.000000000000000000 ) ) ;
#11844=PRODUCT_DEFINITION_SHAPE ( 'NONE', 'NONE',  #1048 ) ;
#11887=TOROIDAL_SURFACE ( 'NONE', #14213, 12.70000000000000284, 0.9000000000000003553 ) ;
#11941=AXIS2_PLACEMENT_3D ( 'NONE', #15063, #12611, #5261 ) ;
#11943=ORIENTED_EDGE ( 'NONE', *, *, #659, .T. ) ;
#11963=AXIS2_PLACEMENT_3D ( 'NONE', #3358, #12963, #17257 ) ;
#11968=AXIS2_PLACEMENT_3D ( 'NONE', #7279, #8816, #15336 ) ;
#11972=VERTEX_POINT ( 'NONE', #7454 ) ;
#12043=SURFACE_SIDE_STYLE ('',( #5148 ) ) ;
#12143=ORIENTED_EDGE ( 'NONE', *, *, #1846, .F. ) ;
#12156=FACE_OUTER_BOUND ( 'NONE', #13732, .T. ) ;
#12168=ORIENTED_EDGE ( 'NONE', *, *, #2101, .F. ) ;
#12188=AXIS2_PLACEMENT_3D ( 'NONE', #3911, #6540, #922 ) ;
#12227=EDGE_CURVE ( 'NONE', #15184, #17384, #5802, .T. ) ;
#12249=DIRECTION ( 'NONE',  ( 1.000000000000000000, 0.000000000000000000, 0.000000000000000000 ) ) ;
#12262=EDGE_CURVE ( 'NONE', #17950, #11972, #4097, .T. ) ;
#12287=ORIENTED_EDGE ( 'NONE', *, *, #16302, .F. ) ;
#12352=ORIENTED_EDGE ( 'NONE', *, *, #16158, .F. ) ;
#12419=DIRECTION ( 'NONE',  ( 1.000000000000000000, 0.000000000000000000, 0.000000000000000000 ) ) ;
#12449=DIRECTION ( 'NONE',  ( -1.000000000000000000, 0.000000000000000000, 0.000000000000000000 ) ) ;
#12455=( NAMED_UNIT ( * ) PLANE_ANGLE_UNIT ( ) SI_UNIT ( $, .RADIAN. ) );
#12463=PRODUCT_DEFINITION_CONTEXT ( 'detailed design', #4811, 'design' ) ;
#12533=CARTESIAN_POINT ( 'NONE',  ( 0.000000000000000000, 0.000000000000000000, -8.722503561260788629 ) ) ;
#12558=EDGE_CURVE ( 'NONE', #17384, #3640, #5539, .T. ) ;
#12597=EDGE_CURVE ( 'NONE', #14976, #6794, #16406, .T. ) ;
#12605=UNCERTAINTY_MEASURE_WITH_UNIT (LENGTH_MEASURE( 1.000000000000000082E-05 ), #13555, 'distance_accuracy_value', 'NONE');
#12611=DIRECTION ( 'NONE',  ( -5.026720092345836698E-22, 4.581671729415424240E-22, -1.000000000000000000 ) ) ;
#12617=DIRECTION ( 'NONE',  ( 0.000000000000000000, 0.000000000000000000, 1.000000000000000000 ) ) ;
#12652=EDGE_CURVE ( 'NONE', #6066, #16345, #11632, .T. ) ;
#12703=AXIS2_PLACEMENT_3D ( 'NONE', #316, #9902, #8470 ) ;
#12717=ADVANCED_FACE ( 'NONE', ( #1706 ), #16290, .F. ) ;
#12747=ORIENTED_EDGE ( 'NONE', *, *, #3011, .T. ) ;
#12768=AXIS2_PLACEMENT_3D ( 'NONE', #4195, #15337, #8539 ) ;
#12782=CIRCLE ( 'NONE', #16271, 10.50000000000000000 ) ;
#12852=CIRCLE ( 'NONE', #1556, 12.50000000000000000 ) ;
#12889=DIRECTION ( 'NONE',  ( 1.000000000000000000, 0.000000000000000000, -0.000000000000000000 ) ) ;
#12906=DIRECTION ( 'NONE',  ( -0.000000000000000000, -0.000000000000000000, -1.000000000000000000 ) ) ;
#12949=ORIENTED_EDGE ( 'NONE', *, *, #8746, .F. ) ;
#12963=DIRECTION ( 'NONE',  ( -5.026720092345836698E-22, 4.581671729415424240E-22, -1.000000000000000000 ) ) ;
#12972=ADVANCED_FACE ( 'NONE', ( #14900 ), #5184, .T. ) ;
#13094=ORIENTED_EDGE ( 'NONE', *, *, #8746, .T. ) ;
#13121=VERTEX_POINT ( 'NONE', #6719 ) ;
#13123=EDGE_CURVE ( 'NONE', #13121, #16345, #2741, .T. ) ;
#13278=CARTESIAN_POINT ( 'NONE',  ( 0.000000000000000000, 0.000000000000000000, -4.000000000000000000 ) ) ;
#13295=DIRECTION ( 'NONE',  ( -0.000000000000000000, -0.000000000000000000, -1.000000000000000000 ) ) ;
#13333=CARTESIAN_POINT ( 'NONE',  ( 12.50000000000000000, 1.530808498934191521E-15, -8.722503561260788629 ) ) ;
#13343=DIRECTION ( 'NONE',  ( 0.9237280213470682178, 0.3830490080632377170, 0.000000000000000000 ) ) ;
#13348=TOROIDAL_SURFACE ( 'NONE', #12768, 12.70000000000000284, 0.9000000000000003553 ) ;
#13349=VERTEX_POINT ( 'NONE', #13333 ) ;
#13360=ORIENTED_EDGE ( 'NONE', *, *, #9666, .T. ) ;
#13364=CARTESIAN_POINT ( 'NONE',  ( 10.47816170930907553, -0.6768509389586216951, -6.005572809000082835 ) ) ;
#13400=LINE ( 'NONE', #16132, #536 ) ;
#13416=DIRECTION ( 'NONE',  ( -0.3830490080632376615, 0.9237280213470682178, 0.000000000000000000 ) ) ;
#13509=( LENGTH_UNIT ( ) NAMED_UNIT ( * ) SI_UNIT ( .MILLI., .METRE. ) );
#13539=EDGE_CURVE ( 'NONE', #17950, #6794, #14998, .T. ) ;
#13541=ORIENTED_EDGE ( 'NONE', *, *, #2690, .T. ) ;
#13555=( LENGTH_UNIT ( ) NAMED_UNIT ( * ) SI_UNIT ( .MILLI., .METRE. ) );
#13559=VECTOR ( 'NONE', #13794, 1000.000000000000000 ) ;
#13612=DIRECTION ( 'NONE',  ( 5.026720092345836698E-22, -4.581671729415424240E-22, 1.000000000000000000 ) ) ;
#13620=APPLICATION_CONTEXT ( 'automotive_design' ) ;
#13661=VECTOR ( 'NONE', #3888, 1000.000000000000000 ) ;
#13691=CIRCLE ( 'NONE', #2684, 11.80000000000000249 ) ;
#13732=EDGE_LOOP ( 'NONE', ( #16085, #7961, #5756, #13541, #16702 ) ) ;
#13759=DIRECTION ( 'NONE',  ( 0.000000000000000000, 0.000000000000000000, 1.000000000000000000 ) ) ;
#13761=DIRECTION ( 'NONE',  ( 0.9237280213470681067, 0.3830490080632377170, 0.000000000000000000 ) ) ;
#13790=DIRECTION ( 'NONE',  ( -5.026720092345836698E-22, 4.581671729415424240E-22, -1.000000000000000000 ) ) ;
#13794=DIRECTION ( 'NONE',  ( -0.000000000000000000, -0.000000000000000000, -1.000000000000000000 ) ) ;
#13886=ORIENTED_EDGE ( 'NONE', *, *, #1937, .F. ) ;
#13930=EDGE_CURVE ( 'NONE', #714, #16745, #15312, .T. ) ;
#13955=ORIENTED_EDGE ( 'NONE', *, *, #13123, .F. ) ;
#13964=AXIS2_PLACEMENT_3D ( 'NONE', #8485, #7135, #333 ) ;
#14072=CARTESIAN_POINT ( 'NONE',  ( -10.50000000000000000, 0.000000000000000000, -7.794427190999915211 ) ) ;
#14213=AXIS2_PLACEMENT_3D ( 'NONE', #15519, #12617, #293 ) ;
#14277=AXIS2_PLACEMENT_3D ( 'NONE', #7569, #10355, #5918 ) ;
#14295=CARTESIAN_POINT ( 'NONE',  ( -12.50000000000000000, 0.000000000000000000, -8.722503561260788629 ) ) ;
#14457=ORIENTED_EDGE ( 'NONE', *, *, #3924, .F. ) ;
#14481=ORIENTED_EDGE ( 'NONE', *, *, #13930, .T. ) ;
#14589=ORIENTED_EDGE ( 'NONE', *, *, #12227, .T. ) ;
#14665=DIRECTION ( 'NONE',  ( 1.000000000000000000, 0.000000000000000000, 0.000000000000000000 ) ) ;
#14705=AXIS2_PLACEMENT_3D ( 'NONE', #13278, #858, #8010 ) ;
#14721=DIRECTION ( 'NONE',  ( -1.000000000000000000, 0.000000000000000000, 0.000000000000000000 ) ) ;
#14734=CARTESIAN_POINT ( 'NONE',  ( 1.296864337298335788E-21, -1.182044466681725685E-21, -6.899999999999998579 ) ) ;
#14742=CIRCLE ( 'NONE', #2009, 11.80000000000000249 ) ;
#14774=EDGE_LOOP ( 'NONE', ( #3606, #3256, #7740, #715, #5636 ) ) ;
#14778=DIRECTION ( 'NONE',  ( -0.9237280213470682178, -0.3830490080632377170, 0.000000000000000000 ) ) ;
#14826=AXIS2_PLACEMENT_3D ( 'NONE', #14734, #17577, #3849 ) ;
#14871=DIRECTION ( 'NONE',  ( 5.026720092345836698E-22, -4.581671729415424240E-22, 1.000000000000000000 ) ) ;
#14883=CYLINDRICAL_SURFACE ( 'NONE', #925, 12.50000000000000000 ) ;
#14900=FACE_OUTER_BOUND ( 'NONE', #15748, .T. ) ;
#14910=ORIENTED_EDGE ( 'NONE', *, *, #6235, .T. ) ;
#14954=DIRECTION ( 'NONE',  ( -1.000000000000000000, 2.131628207280300558E-14, 0.000000000000000000 ) ) ;
#14955=EDGE_CURVE ( 'NONE', #6877, #1158, #3840, .T. ) ;
#14976=VERTEX_POINT ( 'NONE', #2691 ) ;
#14998=CIRCLE ( 'NONE', #17362, 10.50000000000000000 ) ;
#15017=ORIENTED_EDGE ( 'NONE', *, *, #13123, .T. ) ;
#15026=CYLINDRICAL_SURFACE ( 'NONE', #16222, 12.50000000000000000 ) ;
#15036=TOROIDAL_SURFACE ( 'NONE', #1438, 12.70000000000000284, 0.9000000000000003553 ) ;
#15063=CARTESIAN_POINT ( 'NONE',  ( 1.296864337298335788E-21, -1.182044466681725685E-21, -6.899999999999998579 ) ) ;
#15119=DIRECTION ( 'NONE',  ( -0.000000000000000000, -0.000000000000000000, -1.000000000000000000 ) ) ;
#15171=EDGE_LOOP ( 'NONE', ( #5706, #9944, #11442, #12143, #452 ) ) ;
#15184=VERTEX_POINT ( 'NONE', #14295 ) ;
#15280=ADVANCED_FACE ( 'NONE', ( #4491 ), #7224, .F. ) ;
#15309=ORIENTED_EDGE ( 'NONE', *, *, #2471, .F. ) ;
#15312=CIRCLE ( 'NONE', #3750, 10.50000000000000000 ) ;
#15320=AXIS2_PLACEMENT_3D ( 'NONE', #7993, #13790, #6465 ) ;
#15336=DIRECTION ( 'NONE',  ( -1.000000000000000000, 0.000000000000000000, 0.000000000000000000 ) ) ;
#15337=DIRECTION ( 'NONE',  ( 0.000000000000000000, 0.000000000000000000, 1.000000000000000000 ) ) ;
#15356=MECHANICAL_DESIGN_GEOMETRIC_PRESENTATION_REPRESENTATION('',(#599),#9275);
#15368=DIRECTION ( 'NONE',  ( -5.026720092345836698E-22, 4.581671729415424240E-22, -1.000000000000000000 ) ) ;
#15389=CARTESIAN_POINT ( 'NONE',  ( -10.50000000000000000, 0.000000000000000000, -4.000000000000000000 ) ) ;
#15447=ORIENTED_EDGE ( 'NONE', *, *, #6235, .F. ) ;
#15476=VERTEX_POINT ( 'NONE', #15389 ) ;
#15519=CARTESIAN_POINT ( 'NONE',  ( 0.000000000000000000, 0.000000000000000000, -9.600000000000001421 ) ) ;
#15658=VERTEX_POINT ( 'NONE', #5763 ) ;
#15659=CARTESIAN_POINT ( 'NONE',  ( 0.000000000000000000, 0.000000000000000000, -4.000000000000000000 ) ) ;
#15688=DIRECTION ( 'NONE',  ( 0.000000000000000000, 0.000000000000000000, 1.000000000000000000 ) ) ;
#15733=ORIENTED_EDGE ( 'NONE', *, *, #6595, .T. ) ;
#15748=EDGE_LOOP ( 'NONE', ( #17107, #10336 ) ) ;
#15891=FACE_OUTER_BOUND ( 'NONE', #14774, .T. ) ;
#15902=VECTOR ( 'NONE', #17005, 1000.000000000000000 ) ;
#15959=CLOSED_SHELL ( 'NONE', ( #709, #7219, #5953, #2788, #17361, #2623, #629, #1743, #7242, #15280, #12717, #3984, #16979, #17014, #1538, #12972, #6509 ) ) ;
#15970=( NAMED_UNIT ( * ) SI_UNIT ( $, .STERADIAN. ) SOLID_ANGLE_UNIT ( ) );
#16002=ORIENTED_EDGE ( 'NONE', *, *, #3556, .T. ) ;
#16035=CARTESIAN_POINT ( 'NONE',  ( -11.54660026683835383, -4.788112600790469742, -8.722503561260788629 ) ) ;
#16068=FILL_AREA_STYLE_COLOUR ( '', #7273 ) ;
#16085=ORIENTED_EDGE ( 'NONE', *, *, #659, .F. ) ;
#16132=CARTESIAN_POINT ( 'NONE',  ( -10.50000000000000000, 0.000000000000000000, -4.000000000000000000 ) ) ;
#16158=EDGE_CURVE ( 'NONE', #1034, #9766, #16312, .T. ) ;
#16164=DIRECTION ( 'NONE',  ( -0.9979201627913403261, 0.06446199418653535129, 0.000000000000000000 ) ) ;
#16168=CARTESIAN_POINT ( 'NONE',  ( 0.000000000000000000, 0.000000000000000000, -4.000000000000000000 ) ) ;
#16196=DIRECTION ( 'NONE',  ( -0.000000000000000000, -0.000000000000000000, -1.000000000000000000 ) ) ;
#16222=AXIS2_PLACEMENT_3D ( 'NONE', #4057, #15119, #2706 ) ;
#16271=AXIS2_PLACEMENT_3D ( 'NONE', #9423, #9680, #12249 ) ;
#16284=FACE_OUTER_BOUND ( 'NONE', #7979, .T. ) ;
#16290=TOROIDAL_SURFACE ( 'NONE', #11031, 12.70000000000000284, 0.9000000000000003553 ) ;
#16293=FILL_AREA_STYLE_COLOUR ( '', #1469 ) ;
#16296=TOROIDAL_SURFACE ( 'NONE', #11941, 10.40000000000000036, 0.9000000000000003553 ) ;
#16302=EDGE_CURVE ( 'NONE', #6794, #15658, #964, .T. ) ;
#16310=AXIS2_PLACEMENT_3D ( 'NONE', #16899, #7375, #12889 ) ;
#16312=CIRCLE ( 'NONE', #5554, 12.50000000000000000 ) ;
#16332=SHAPE_REPRESENTATION ( 'ceramic piston', ( #3575 ), #3784 ) ;
#16345=VERTEX_POINT ( 'NONE', #11638 ) ;
#16356=CYLINDRICAL_SURFACE ( 'NONE', #3430, 10.50000000000000000 ) ;
#16405=FACE_OUTER_BOUND ( 'NONE', #1475, .T. ) ;
#16406=LINE ( 'NONE', #10498, #13661 ) ;
#16486=DIRECTION ( 'NONE',  ( 0.000000000000000000, 0.000000000000000000, 1.000000000000000000 ) ) ;
#16493=CIRCLE ( 'NONE', #1172, 12.50000000000000000 ) ;
#16512=DIRECTION ( 'NONE',  ( -1.000000000000000000, 0.000000000000000000, 0.000000000000000000 ) ) ;
#16518=DIRECTION ( 'NONE',  ( -1.000000000000000000, 0.000000000000000000, 0.000000000000000000 ) ) ;
#16630=EDGE_CURVE ( 'NONE', #13349, #6877, #12852, .T. ) ;
#16702=ORIENTED_EDGE ( 'NONE', *, *, #9180, .F. ) ;
#16731=DIRECTION ( 'NONE',  ( -0.000000000000000000, -0.000000000000000000, -1.000000000000000000 ) ) ;
#16745=VERTEX_POINT ( 'NONE', #4495 ) ;
#16757=DIRECTION ( 'NONE',  ( 1.000000000000000000, 0.000000000000000000, 0.000000000000000000 ) ) ;
#16821=FACE_OUTER_BOUND ( 'NONE', #9672, .T. ) ;
#16850=ORIENTED_EDGE ( 'NONE', *, *, #2146, .F. ) ;
#16899=CARTESIAN_POINT ( 'NONE',  ( 0.000000000000000000, 0.000000000000000000, -4.000000000000000000 ) ) ;
#16901=VERTEX_POINT ( 'NONE', #11057 ) ;
#16928=DIRECTION ( 'NONE',  ( -0.000000000000000000, -0.000000000000000000, -1.000000000000000000 ) ) ;
#16929=SHAPE_DEFINITION_REPRESENTATION ( #11844, #16332 ) ;
#16979=ADVANCED_FACE ( 'NONE', ( #17077, #8725 ), #4630, .T. ) ;
#16993=VERTEX_POINT ( 'NONE', #11506 ) ;
#17005=DIRECTION ( 'NONE',  ( -0.000000000000000000, -0.000000000000000000, -1.000000000000000000 ) ) ;
#17014=ADVANCED_FACE ( 'NONE', ( #3285 ), #8625, .F. ) ;
#17063=CARTESIAN_POINT ( 'NONE',  ( 12.50000000000000000, 1.530808498934191521E-15, -4.000000000000000000 ) ) ;
#17077=FACE_BOUND ( 'NONE', #7880, .T. ) ;
#17078=VERTEX_POINT ( 'NONE', #9879 ) ;
#17079=CIRCLE ( 'NONE', #17682, 12.50000000000000000 ) ;
#17086=ORIENTED_EDGE ( 'NONE', *, *, #3924, .T. ) ;
#17103=ORIENTED_EDGE ( 'NONE', *, *, #13539, .T. ) ;
#17107=ORIENTED_EDGE ( 'NONE', *, *, #12652, .T. ) ;
#17194=ORIENTED_EDGE ( 'NONE', *, *, #12597, .F. ) ;
#17257=DIRECTION ( 'NONE',  ( 1.000000000000000000, 0.000000000000000000, 0.000000000000000000 ) ) ;
#17294=ORIENTED_EDGE ( 'NONE', *, *, #16630, .F. ) ;
#17309=ORIENTED_EDGE ( 'NONE', *, *, #7263, .F. ) ;
#17337=VECTOR ( 'NONE', #12906, 1000.000000000000000 ) ;
#17361=ADVANCED_FACE ( 'NONE', ( #6030 ), #10380, .F. ) ;
#17362=AXIS2_PLACEMENT_3D ( 'NONE', #10589, #14871, #14954 ) ;
#17381=LINE ( 'NONE', #11630, #17337 ) ;
#17384=VERTEX_POINT ( 'NONE', #16035 ) ;
#17468=AXIS2_PLACEMENT_3D ( 'NONE', #10659, #13416, #14778 ) ;
#17508=AXIS2_PLACEMENT_3D ( 'NONE', #4924, #2230, #7744 ) ;
#17509=ORIENTED_EDGE ( 'NONE', *, *, #12262, .T. ) ;
#17575=DIRECTION ( 'NONE',  ( 0.000000000000000000, 0.000000000000000000, 1.000000000000000000 ) ) ;
#17577=DIRECTION ( 'NONE',  ( -5.026720092345836698E-22, 4.581671729415424240E-22, -1.000000000000000000 ) ) ;
#17597=LINE ( 'NONE', #5116, #7541 ) ;
#17608=DIRECTION ( 'NONE',  ( -0.000000000000000000, -0.000000000000000000, -1.000000000000000000 ) ) ;
#17650=CARTESIAN_POINT ( 'NONE',  ( 0.000000000000000000, 0.000000000000000000, -4.000000000000000000 ) ) ;
#17656=ORIENTED_EDGE ( 'NONE', *, *, #9180, .T. ) ;
#17660=ORIENTED_EDGE ( 'NONE', *, *, #8457, .F. ) ;
#17662=DIRECTION ( 'NONE',  ( 1.000000000000000000, 0.000000000000000000, -0.000000000000000000 ) ) ;
#17682=AXIS2_PLACEMENT_3D ( 'NONE', #1897, #4424, #524 ) ;
#17706=DIRECTION ( 'NONE',  ( -0.9237280213470682178, -0.3830490080632377170, 0.000000000000000000 ) ) ;
#17745=AXIS2_PLACEMENT_3D ( 'NONE', #6457, #5160, #16164 ) ;
#17773=EDGE_CURVE ( 'NONE', #15658, #16745, #6731, .T. ) ;
#17876=DIRECTION ( 'NONE',  ( 0.000000000000000000, 0.000000000000000000, 1.000000000000000000 ) ) ;
#17931=PRESENTATION_STYLE_ASSIGNMENT (( #2764 ) ) ;
#17950=VERTEX_POINT ( 'NONE', #13364 ) ;
ENDSEC;
END-ISO-10303-21;
